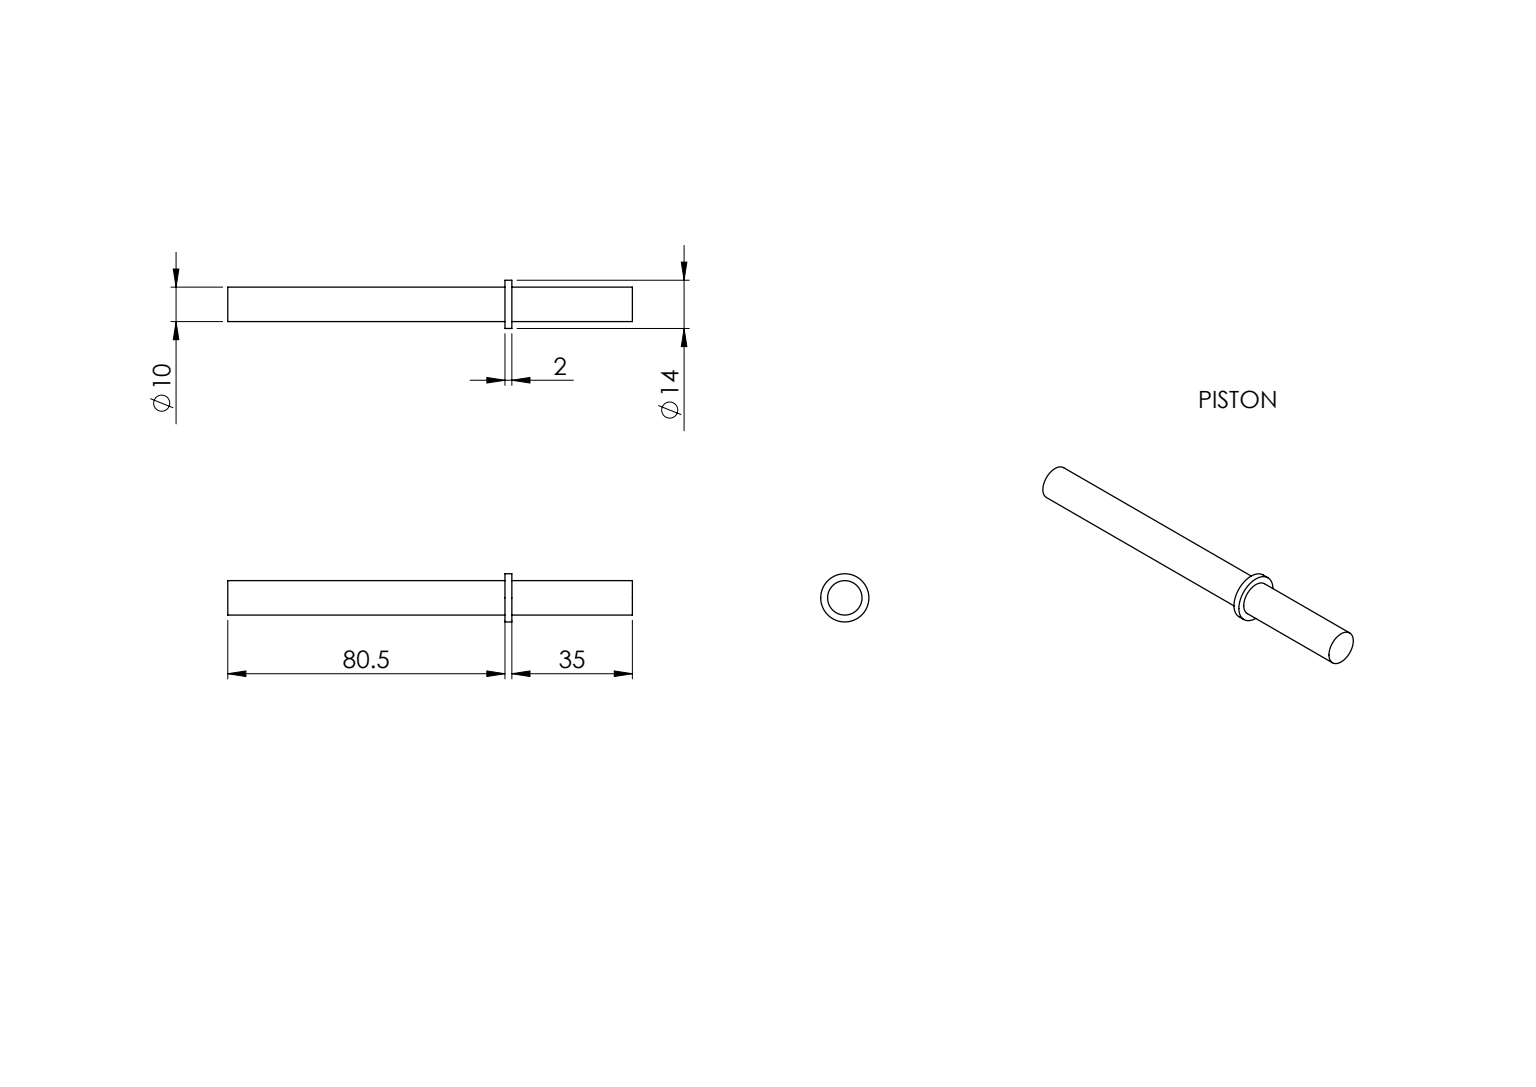
ISO-10303-21;
HEADER;
FILE_DESCRIPTION (('STEP AP214'),
    '1' );
FILE_NAME ('piston.step',
    '2026-10-27T14:18:53',
    ( '' ),
    ( '' ),
    'SwSTEP 2.0',
    'SolidWorks 2026',
    '' );
FILE_SCHEMA (( 'AUTOMOTIVE_DESIGN' ));
ENDSEC;

DATA;
#2=PLANE ( 'NONE',  #2825 ) ;
#50=DIRECTION ( 'NONE',  ( -1.000000000000000000, -0.000000000000000000, -0.000000000000000000 ) ) ;
#53=( NAMED_UNIT ( * ) PLANE_ANGLE_UNIT ( ) SI_UNIT ( $, .RADIAN. ) );
#122=CARTESIAN_POINT ( 'NONE',  ( 135.4999999999999716, 0.000000000000000000, 0.000000000000000000 ) ) ;
#126=MANIFOLD_SOLID_BREP ( 'Boss-Extrude2', #2558 ) ;
#155=ORIENTED_EDGE ( 'NONE', *, *, #5293, .T. ) ;
#159=EDGE_CURVE ( 'NONE', #4312, #626, #169, .T. ) ;
#169=LINE ( 'NONE', #5681, #675 ) ;
#172=DIRECTION ( 'NONE',  ( 0.000000000000000000, 0.000000000000000000, -1.000000000000000000 ) ) ;
#214=CARTESIAN_POINT ( 'NONE',  ( 137.4999999999999716, 0.000000000000000000, 5.000000000000000000 ) ) ;
#218=AXIS2_PLACEMENT_3D ( 'NONE', #3417, #2963, #2469 ) ;
#223=AXIS2_PLACEMENT_3D ( 'NONE', #4631, #50, #5962 ) ;
#241=SHAPE_DEFINITION_REPRESENTATION ( #544, #4225 ) ;
#261=ORIENTED_EDGE ( 'NONE', *, *, #932, .T. ) ;
#264=DIRECTION ( 'NONE',  ( -1.000000000000000000, -0.000000000000000000, -0.000000000000000000 ) ) ;
#265=ORIENTED_EDGE ( 'NONE', *, *, #3879, .F. ) ;
#267=CARTESIAN_POINT ( 'NONE',  ( 196.6421356237309510, 0.000000000000000000, 5.000000000000000000 ) ) ;
#289=DIRECTION ( 'NONE',  ( 0.000000000000000000, 0.000000000000000000, 1.000000000000000000 ) ) ;
#334=ADVANCED_FACE ( 'NONE', ( #4537 ), #4626, .F. ) ;
#384=ORIENTED_EDGE ( 'NONE', *, *, #5078, .T. ) ;
#395=EDGE_LOOP ( 'NONE', ( #4054, #2100 ) ) ;
#411=VECTOR ( 'NONE', #264, 1000.000000000000000 ) ;
#430=( LENGTH_UNIT ( ) NAMED_UNIT ( * ) SI_UNIT ( .MILLI., .METRE. ) );
#451=PLANE ( 'NONE',  #1857 ) ;
#456=VECTOR ( 'NONE', #5335, 1000.000000000000000 ) ;
#462=CARTESIAN_POINT ( 'NONE',  ( 172.5000000000000284, 15.00000000000000000, 75.00000000000001421 ) ) ;
#466=DIRECTION ( 'NONE',  ( -1.000000000000000000, 0.000000000000000000, 0.000000000000000000 ) ) ;
#478=CARTESIAN_POINT ( 'NONE',  ( 55.00000000000000711, 0.000000000000000000, 5.000000000000000000 ) ) ;
#544=PRODUCT_DEFINITION_SHAPE ( 'NONE', 'NONE',  #3311 ) ;
#575=AXIS2_PLACEMENT_3D ( 'NONE', #1998, #3850, #3404 ) ;
#590=AXIS2_PLACEMENT_3D ( 'NONE', #4311, #4369, #5694 ) ;
#626=VERTEX_POINT ( 'NONE', #3463 ) ;
#647=ORIENTED_EDGE ( 'NONE', *, *, #1643, .T. ) ;
#663=AXIS2_PLACEMENT_3D ( 'NONE', #4941, #4491, #775 ) ;
#667=DIRECTION ( 'NONE',  ( 1.000000000000000000, 0.000000000000000000, 0.000000000000000000 ) ) ;
#675=VECTOR ( 'NONE', #3854, 1000.000000000000000 ) ;
#676=AXIS2_PLACEMENT_3D ( 'NONE', #3452, #3515, #5369 ) ;
#749=CARTESIAN_POINT ( 'NONE',  ( 137.4999999999999716, 8.572527594031473190E-16, 7.000000000000000000 ) ) ;
#775=DIRECTION ( 'NONE',  ( 0.000000000000000000, 0.000000000000000000, -1.000000000000000000 ) ) ;
#780=DIRECTION ( 'NONE',  ( 1.000000000000000000, -0.000000000000000000, -0.000000000000000000 ) ) ;
#795=VECTOR ( 'NONE', #780, 1000.000000000000000 ) ;
#810=ADVANCED_FACE ( 'NONE', ( #4064 ), #3617, .T. ) ;
#817=( NAMED_UNIT ( * ) PLANE_ANGLE_UNIT ( ) SI_UNIT ( $, .RADIAN. ) );
#852=ORIENTED_EDGE ( 'NONE', *, *, #5084, .T. ) ;
#873=CYLINDRICAL_SURFACE ( 'NONE', #5492, 7.000000000000000000 ) ;
#920=FACE_OUTER_BOUND ( 'NONE', #5008, .T. ) ;
#926=AXIS2_PLACEMENT_3D ( 'NONE', #3342, #2851, #4711 ) ;
#927=FACE_OUTER_BOUND ( 'NONE', #3682, .T. ) ;
#932=EDGE_CURVE ( 'NONE', #3440, #5157, #3043, .T. ) ;
#936=EDGE_LOOP ( 'NONE', ( #4735, #3724 ) ) ;
#953=CARTESIAN_POINT ( 'NONE',  ( 55.00000000000000711, 0.000000000000000000, 0.000000000000000000 ) ) ;
#961=( GEOMETRIC_REPRESENTATION_CONTEXT ( 3 ) GLOBAL_UNCERTAINTY_ASSIGNED_CONTEXT ( ( #1965 ) ) GLOBAL_UNIT_ASSIGNED_CONTEXT ( ( #2755, #53, #2314 ) ) REPRESENTATION_CONTEXT ( 'NONE', 'WORKASPACE' ) );
#976=EDGE_CURVE ( 'NONE', #626, #5459, #5968, .T. ) ;
#983=AXIS2_PLACEMENT_3D ( 'NONE', #5013, #5074, #3743 ) ;
#1135=CARTESIAN_POINT ( 'NONE',  ( 135.4999999999999716, 0.000000000000000000, 5.000000000000000000 ) ) ;
#1138=ORIENTED_EDGE ( 'NONE', *, *, #976, .T. ) ;
#1149=EDGE_LOOP ( 'NONE', ( #265, #5106 ) ) ;
#1172=CIRCLE ( 'NONE', #218, 5.000000000000000000 ) ;
#1176=( LENGTH_UNIT ( ) NAMED_UNIT ( * ) SI_UNIT ( .MILLI., .METRE. ) );
#1185=STYLED_ITEM ( 'NONE', ( #4986 ), #3198 ) ;
#1251=EDGE_LOOP ( 'NONE', ( #5497, #155, #2860, #3324 ) ) ;
#1262=UNCERTAINTY_MEASURE_WITH_UNIT (LENGTH_MEASURE( 1.000000000000000082E-05 ), #1176, 'distance_accuracy_value', 'NONE');
#1265=ORIENTED_EDGE ( 'NONE', *, *, #5682, .T. ) ;
#1285=ORIENTED_EDGE ( 'NONE', *, *, #1568, .F. ) ;
#1305=CARTESIAN_POINT ( 'NONE',  ( 135.4999999999999716, 0.000000000000000000, 0.000000000000000000 ) ) ;
#1310=ORIENTED_EDGE ( 'NONE', *, *, #5372, .T. ) ;
#1320=ADVANCED_FACE ( 'NONE', ( #5046 ), #873, .T. ) ;
#1327=VERTEX_POINT ( 'NONE', #478 ) ;
#1332=CARTESIAN_POINT ( 'NONE',  ( 172.5000000000000284, 0.000000000000000000, 5.000000000000000000 ) ) ;
#1402=CYLINDRICAL_SURFACE ( 'NONE', #4867, 5.000000000000000000 ) ;
#1446=AXIS2_PLACEMENT_3D ( 'NONE', #3748, #3337, #5692 ) ;
#1460=VECTOR ( 'NONE', #4573, 1000.000000000000000 ) ;
#1469=CARTESIAN_POINT ( 'NONE',  ( 135.4999999999999716, 0.000000000000000000, 0.000000000000000000 ) ) ;
#1525=DIRECTION ( 'NONE',  ( 1.000000000000000000, 0.000000000000000000, 0.000000000000000000 ) ) ;
#1568=EDGE_CURVE ( 'NONE', #2772, #5459, #5846, .T. ) ;
#1593=CARTESIAN_POINT ( 'NONE',  ( 137.4999999999999716, 0.000000000000000000, -7.000000000000000000 ) ) ;
#1639=ORIENTED_EDGE ( 'NONE', *, *, #2435, .T. ) ;
#1643=EDGE_CURVE ( 'NONE', #1327, #4518, #3174, .T. ) ;
#1728=DIRECTION ( 'NONE',  ( 0.000000000000000000, 0.000000000000000000, -1.000000000000000000 ) ) ;
#1800=DIRECTION ( 'NONE',  ( 0.000000000000000000, 0.000000000000000000, 1.000000000000000000 ) ) ;
#1809=FACE_OUTER_BOUND ( 'NONE', #395, .T. ) ;
#1857=AXIS2_PLACEMENT_3D ( 'NONE', #953, #2320, #2380 ) ;
#1867=DIRECTION ( 'NONE',  ( 0.000000000000000000, 0.000000000000000000, 1.000000000000000000 ) ) ;
#1885=CARTESIAN_POINT ( 'NONE',  ( 172.5000000000000284, 0.000000000000000000, 0.000000000000000000 ) ) ;
#1956=MECHANICAL_DESIGN_GEOMETRIC_PRESENTATION_REPRESENTATION('',(#1185),#4684);
#1965=UNCERTAINTY_MEASURE_WITH_UNIT (LENGTH_MEASURE( 1.000000000000000082E-05 ), #2755, 'distance_accuracy_value', 'NONE');
#1998=CARTESIAN_POINT ( 'NONE',  ( 137.4999999999999716, 0.000000000000000000, 0.000000000000000000 ) ) ;
#2001=ORIENTED_EDGE ( 'NONE', *, *, #5660, .F. ) ;
#2015=PLANE ( 'NONE',  #676 ) ;
#2023=( NAMED_UNIT ( * ) SI_UNIT ( $, .STERADIAN. ) SOLID_ANGLE_UNIT ( ) );
#2100=ORIENTED_EDGE ( 'NONE', *, *, #3397, .F. ) ;
#2142=FACE_OUTER_BOUND ( 'NONE', #1251, .T. ) ;
#2147=( NAMED_UNIT ( * ) SI_UNIT ( $, .STERADIAN. ) SOLID_ANGLE_UNIT ( ) );
#2149=AXIS2_PLACEMENT_3D ( 'NONE', #4002, #5456, #3158 ) ;
#2171=LINE ( 'NONE', #4021, #1460 ) ;
#2198=DIRECTION ( 'NONE',  ( -1.000000000000000000, 0.000000000000000000, 0.000000000000000000 ) ) ;
#2217=DIRECTION ( 'NONE',  ( 0.000000000000000000, 0.000000000000000000, 1.000000000000000000 ) ) ;
#2226=EDGE_LOOP ( 'NONE', ( #852, #1310, #3329, #3767 ) ) ;
#2242=AXIS2_PLACEMENT_3D ( 'NONE', #122, #2540, #4341 ) ;
#2290=DIRECTION ( 'NONE',  ( 0.000000000000000000, 0.000000000000000000, 1.000000000000000000 ) ) ;
#2311=FACE_OUTER_BOUND ( 'NONE', #5227, .T. ) ;
#2312=VERTEX_POINT ( 'NONE', #4606 ) ;
#2314=( NAMED_UNIT ( * ) SI_UNIT ( $, .STERADIAN. ) SOLID_ANGLE_UNIT ( ) );
#2320=DIRECTION ( 'NONE',  ( 1.000000000000000000, 0.000000000000000000, 0.000000000000000000 ) ) ;
#2380=DIRECTION ( 'NONE',  ( 0.000000000000000000, 0.000000000000000000, -1.000000000000000000 ) ) ;
#2383=ORIENTED_EDGE ( 'NONE', *, *, #5393, .F. ) ;
#2435=EDGE_CURVE ( 'NONE', #5618, #3394, #3004, .T. ) ;
#2454=DIRECTION ( 'NONE',  ( -1.000000000000000000, 0.000000000000000000, 0.000000000000000000 ) ) ;
#2457=ORIENTED_EDGE ( 'NONE', *, *, #4055, .T. ) ;
#2469=DIRECTION ( 'NONE',  ( 0.000000000000000000, 0.000000000000000000, 1.000000000000000000 ) ) ;
#2503=ORIENTED_EDGE ( 'NONE', *, *, #932, .F. ) ;
#2526=CARTESIAN_POINT ( 'NONE',  ( 55.00000000000000711, 0.000000000000000000, 0.000000000000000000 ) ) ;
#2531=CARTESIAN_POINT ( 'NONE',  ( 135.4999999999999716, 0.000000000000000000, -7.000000000000000000 ) ) ;
#2534=PRODUCT_CONTEXT ( 'NONE', #2846, 'mechanical' ) ;
#2540=DIRECTION ( 'NONE',  ( -1.000000000000000000, 0.000000000000000000, 0.000000000000000000 ) ) ;
#2558=CLOSED_SHELL ( 'NONE', ( #4050, #810, #2681, #5719, #4047, #1320, #5759, #2881, #334, #5678 ) ) ;
#2599=SURFACE_STYLE_FILL_AREA ( #4527 ) ;
#2617=CARTESIAN_POINT ( 'NONE',  ( 135.4999999999999716, 8.572527594031473190E-16, 7.000000000000000000 ) ) ;
#2637=DIRECTION ( 'NONE',  ( 1.000000000000000000, -0.000000000000000000, -0.000000000000000000 ) ) ;
#2681=ADVANCED_FACE ( 'NONE', ( #5662 ), #5954, .T. ) ;
#2743=AXIS2_PLACEMENT_3D ( 'NONE', #1305, #3165, #1728 ) ;
#2755=( LENGTH_UNIT ( ) NAMED_UNIT ( * ) SI_UNIT ( .MILLI., .METRE. ) );
#2772=VERTEX_POINT ( 'NONE', #1332 ) ;
#2802=EDGE_LOOP ( 'NONE', ( #3718, #1138 ) ) ;
#2809=FACE_BOUND ( 'NONE', #3116, .T. ) ;
#2825=AXIS2_PLACEMENT_3D ( 'NONE', #1469, #4151, #1867 ) ;
#2827=AXIS2_PLACEMENT_3D ( 'NONE', #4019, #4422, #289 ) ;
#2846=APPLICATION_CONTEXT ( 'automotive_design' ) ;
#2851=DIRECTION ( 'NONE',  ( -1.000000000000000000, 0.000000000000000000, 0.000000000000000000 ) ) ;
#2860=ORIENTED_EDGE ( 'NONE', *, *, #1568, .T. ) ;
#2881=ADVANCED_FACE ( 'NONE', ( #5338, #2968 ), #2015, .F. ) ;
#2949=VERTEX_POINT ( 'NONE', #1135 ) ;
#2963=DIRECTION ( 'NONE',  ( -1.000000000000000000, 0.000000000000000000, 0.000000000000000000 ) ) ;
#2968=FACE_OUTER_BOUND ( 'NONE', #1149, .T. ) ;
#3004=CIRCLE ( 'NONE', #575, 7.000000000000000000 ) ;
#3039=( GEOMETRIC_REPRESENTATION_CONTEXT ( 3 ) GLOBAL_UNCERTAINTY_ASSIGNED_CONTEXT ( ( #1262 ) ) GLOBAL_UNIT_ASSIGNED_CONTEXT ( ( #1176, #3521, #2023 ) ) REPRESENTATION_CONTEXT ( 'NONE', 'WORKASPACE' ) );
#3040=ORIENTED_EDGE ( 'NONE', *, *, #5426, .T. ) ;
#3043=CIRCLE ( 'NONE', #5277, 7.000000000000000000 ) ;
#3087=UNCERTAINTY_MEASURE_WITH_UNIT (LENGTH_MEASURE( 1.000000000000000082E-05 ), #430, 'distance_accuracy_value', 'NONE');
#3093=SURFACE_SIDE_STYLE ('',( #2599 ) ) ;
#3116=EDGE_LOOP ( 'NONE', ( #3340, #4294 ) ) ;
#3118=VECTOR ( 'NONE', #5066, 1000.000000000000000 ) ;
#3158=DIRECTION ( 'NONE',  ( 0.000000000000000000, 0.000000000000000000, 1.000000000000000000 ) ) ;
#3165=DIRECTION ( 'NONE',  ( 1.000000000000000000, -0.000000000000000000, -0.000000000000000000 ) ) ;
#3174=CIRCLE ( 'NONE', #663, 5.000000000000000000 ) ;
#3187=CARTESIAN_POINT ( 'NONE',  ( 135.4999999999999716, 0.000000000000000000, -7.000000000000000000 ) ) ;
#3191=SHAPE_REPRESENTATION_RELATIONSHIP ( 'NONE' , 'NONE' ,  #4225, #3198 ) ;
#3198=ADVANCED_BREP_SHAPE_REPRESENTATION ( '', ( #126, #5080 ), #3039 ) ;
#3207=CYLINDRICAL_SURFACE ( 'NONE', #223, 5.000000000000000000 ) ;
#3210=CARTESIAN_POINT ( 'NONE',  ( 135.4999999999999716, 8.572527594031473190E-16, 7.000000000000000000 ) ) ;
#3222=FILL_AREA_STYLE_COLOUR ( '', #4202 ) ;
#3264=ORIENTED_EDGE ( 'NONE', *, *, #5393, .T. ) ;
#3311=PRODUCT_DEFINITION ( 'UNKNOWN', '', #4599, #5937 ) ;
#3324=ORIENTED_EDGE ( 'NONE', *, *, #976, .F. ) ;
#3329=ORIENTED_EDGE ( 'NONE', *, *, #3397, .T. ) ;
#3337=DIRECTION ( 'NONE',  ( -1.000000000000000000, -0.000000000000000000, -0.000000000000000000 ) ) ;
#3340=ORIENTED_EDGE ( 'NONE', *, *, #5084, .F. ) ;
#3342=CARTESIAN_POINT ( 'NONE',  ( 137.4999999999999716, 0.000000000000000000, 0.000000000000000000 ) ) ;
#3352=ORIENTED_EDGE ( 'NONE', *, *, #3879, .T. ) ;
#3394=VERTEX_POINT ( 'NONE', #1593 ) ;
#3397=EDGE_CURVE ( 'NONE', #4518, #1327, #5153, .T. ) ;
#3404=DIRECTION ( 'NONE',  ( 0.000000000000000000, 0.000000000000000000, 1.000000000000000000 ) ) ;
#3414=EDGE_LOOP ( 'NONE', ( #2503, #3264, #1639, #2001 ) ) ;
#3417=CARTESIAN_POINT ( 'NONE',  ( 135.4999999999999716, 0.000000000000000000, 0.000000000000000000 ) ) ;
#3440=VERTEX_POINT ( 'NONE', #2617 ) ;
#3452=CARTESIAN_POINT ( 'NONE',  ( 137.4999999999999716, 0.000000000000000000, 0.000000000000000000 ) ) ;
#3463=CARTESIAN_POINT ( 'NONE',  ( 137.4999999999999716, 6.123233995736766282E-16, -5.000000000000000000 ) ) ;
#3515=DIRECTION ( 'NONE',  ( -1.000000000000000000, 0.000000000000000000, 0.000000000000000000 ) ) ;
#3521=( NAMED_UNIT ( * ) PLANE_ANGLE_UNIT ( ) SI_UNIT ( $, .RADIAN. ) );
#3527=CARTESIAN_POINT ( 'NONE',  ( 0.000000000000000000, 0.000000000000000000, 0.000000000000000000 ) ) ;
#3617=CYLINDRICAL_SURFACE ( 'NONE', #2743, 7.000000000000000000 ) ;
#3631=CARTESIAN_POINT ( 'NONE',  ( 172.5000000000000284, 0.000000000000000000, 0.000000000000000000 ) ) ;
#3657=LINE ( 'NONE', #3210, #3118 ) ;
#3682=EDGE_LOOP ( 'NONE', ( #1265, #261 ) ) ;
#3699=AXIS2_PLACEMENT_3D ( 'NONE', #3631, #2198, #4543 ) ;
#3718=ORIENTED_EDGE ( 'NONE', *, *, #4697, .T. ) ;
#3724=ORIENTED_EDGE ( 'NONE', *, *, #5293, .F. ) ;
#3743=DIRECTION ( 'NONE',  ( 0.000000000000000000, 0.000000000000000000, 1.000000000000000000 ) ) ;
#3748=CARTESIAN_POINT ( 'NONE',  ( 196.6421356237309510, 0.000000000000000000, 0.000000000000000000 ) ) ;
#3749=CARTESIAN_POINT ( 'NONE',  ( 55.00000000000000711, 6.123233995736766282E-16, -5.000000000000000000 ) ) ;
#3767=ORIENTED_EDGE ( 'NONE', *, *, #5078, .F. ) ;
#3787=CIRCLE ( 'NONE', #4771, 5.000000000000000000 ) ;
#3799=ORIENTED_EDGE ( 'NONE', *, *, #4697, .F. ) ;
#3850=DIRECTION ( 'NONE',  ( -1.000000000000000000, 0.000000000000000000, 0.000000000000000000 ) ) ;
#3854=DIRECTION ( 'NONE',  ( -1.000000000000000000, -0.000000000000000000, -0.000000000000000000 ) ) ;
#3879=EDGE_CURVE ( 'NONE', #3394, #5618, #4192, .T. ) ;
#3986=ORIENTED_EDGE ( 'NONE', *, *, #5682, .F. ) ;
#4002=CARTESIAN_POINT ( 'NONE',  ( 196.6421356237309510, 0.000000000000000000, 0.000000000000000000 ) ) ;
#4019=CARTESIAN_POINT ( 'NONE',  ( 137.4999999999999716, 0.000000000000000000, 0.000000000000000000 ) ) ;
#4021=CARTESIAN_POINT ( 'NONE',  ( 196.6421356237309510, 6.123233995736766282E-16, -5.000000000000000000 ) ) ;
#4047=ADVANCED_FACE ( 'NONE', ( #2311 ), #3207, .T. ) ;
#4050=ADVANCED_FACE ( 'NONE', ( #920 ), #1402, .T. ) ;
#4054=ORIENTED_EDGE ( 'NONE', *, *, #1643, .F. ) ;
#4055=EDGE_CURVE ( 'NONE', #2772, #4312, #3787, .T. ) ;
#4064=FACE_OUTER_BOUND ( 'NONE', #3414, .T. ) ;
#4078=CIRCLE ( 'NONE', #590, 5.000000000000000000 ) ;
#4099=EDGE_LOOP ( 'NONE', ( #2383, #3986, #5294, #3352 ) ) ;
#4151=DIRECTION ( 'NONE',  ( -1.000000000000000000, 0.000000000000000000, 0.000000000000000000 ) ) ;
#4192=CIRCLE ( 'NONE', #2827, 7.000000000000000000 ) ;
#4202=COLOUR_RGB ( '',0.8941176470588234615, 0.8941176470588234615, 0.8941176470588234615 ) ;
#4208=AXIS2_PLACEMENT_3D ( 'NONE', #462, #5557, #2217 ) ;
#4225=SHAPE_REPRESENTATION ( 'piston', ( #5080 ), #3039 ) ;
#4294=ORIENTED_EDGE ( 'NONE', *, *, #5426, .F. ) ;
#4311=CARTESIAN_POINT ( 'NONE',  ( 137.4999999999999716, 0.000000000000000000, 0.000000000000000000 ) ) ;
#4312=VERTEX_POINT ( 'NONE', #5909 ) ;
#4341=DIRECTION ( 'NONE',  ( 0.000000000000000000, 0.000000000000000000, 1.000000000000000000 ) ) ;
#4369=DIRECTION ( 'NONE',  ( -1.000000000000000000, 0.000000000000000000, 0.000000000000000000 ) ) ;
#4422=DIRECTION ( 'NONE',  ( -1.000000000000000000, 0.000000000000000000, 0.000000000000000000 ) ) ;
#4467=MECHANICAL_DESIGN_GEOMETRIC_PRESENTATION_REPRESENTATION('',(#4950),#961);
#4491=DIRECTION ( 'NONE',  ( 1.000000000000000000, 0.000000000000000000, 0.000000000000000000 ) ) ;
#4495=LINE ( 'NONE', #3187, #795 ) ;
#4499=DIRECTION ( 'NONE',  ( 0.000000000000000000, 0.000000000000000000, -1.000000000000000000 ) ) ;
#4518=VERTEX_POINT ( 'NONE', #3749 ) ;
#4527=FILL_AREA_STYLE ('',( #3222 ) ) ;
#4537=FACE_OUTER_BOUND ( 'NONE', #936, .T. ) ;
#4543=DIRECTION ( 'NONE',  ( 0.000000000000000000, 0.000000000000000000, 1.000000000000000000 ) ) ;
#4573=DIRECTION ( 'NONE',  ( -1.000000000000000000, -0.000000000000000000, -0.000000000000000000 ) ) ;
#4599=PRODUCT_DEFINITION_FORMATION_WITH_SPECIFIED_SOURCE ( 'ANY', '', #4847, .NOT_KNOWN. ) ;
#4606=CARTESIAN_POINT ( 'NONE',  ( 135.4999999999999716, 6.123233995736766282E-16, -5.000000000000000000 ) ) ;
#4626=PLANE ( 'NONE',  #4208 ) ;
#4631=CARTESIAN_POINT ( 'NONE',  ( 196.6421356237309510, 0.000000000000000000, 0.000000000000000000 ) ) ;
#4672=CIRCLE ( 'NONE', #2242, 5.000000000000000000 ) ;
#4681=CARTESIAN_POINT ( 'NONE',  ( 135.4999999999999716, 0.000000000000000000, 0.000000000000000000 ) ) ;
#4684=( GEOMETRIC_REPRESENTATION_CONTEXT ( 3 ) GLOBAL_UNCERTAINTY_ASSIGNED_CONTEXT ( ( #3087 ) ) GLOBAL_UNIT_ASSIGNED_CONTEXT ( ( #430, #817, #2147 ) ) REPRESENTATION_CONTEXT ( 'NONE', 'WORKASPACE' ) );
#4697=EDGE_CURVE ( 'NONE', #5459, #626, #4078, .T. ) ;
#4711=DIRECTION ( 'NONE',  ( 0.000000000000000000, 0.000000000000000000, 1.000000000000000000 ) ) ;
#4735=ORIENTED_EDGE ( 'NONE', *, *, #4055, .F. ) ;
#4753=LINE ( 'NONE', #4883, #411 ) ;
#4769=CIRCLE ( 'NONE', #3699, 5.000000000000000000 ) ;
#4771=AXIS2_PLACEMENT_3D ( 'NONE', #1885, #466, #1800 ) ;
#4831=DIRECTION ( 'NONE',  ( 0.000000000000000000, 0.000000000000000000, 1.000000000000000000 ) ) ;
#4847=PRODUCT ( 'piston', 'piston', '', ( #2534 ) ) ;
#4867=AXIS2_PLACEMENT_3D ( 'NONE', #5093, #5145, #2290 ) ;
#4883=CARTESIAN_POINT ( 'NONE',  ( 196.6421356237309510, 0.000000000000000000, 5.000000000000000000 ) ) ;
#4935=ORIENTED_EDGE ( 'NONE', *, *, #5372, .F. ) ;
#4941=CARTESIAN_POINT ( 'NONE',  ( 55.00000000000000711, 0.000000000000000000, 0.000000000000000000 ) ) ;
#4943=APPLICATION_CONTEXT ( 'automotive_design' ) ;
#4950=STYLED_ITEM('',(#6013),#126);
#4986=PRESENTATION_STYLE_ASSIGNMENT (( #5045 ) ) ;
#5008=EDGE_LOOP ( 'NONE', ( #2457, #5580, #3799, #1285 ) ) ;
#5013=CARTESIAN_POINT ( 'NONE',  ( 135.4999999999999716, 0.000000000000000000, 0.000000000000000000 ) ) ;
#5045=SURFACE_STYLE_USAGE ( .BOTH. , #3093 ) ;
#5046=FACE_OUTER_BOUND ( 'NONE', #4099, .T. ) ;
#5066=DIRECTION ( 'NONE',  ( 1.000000000000000000, -0.000000000000000000, -0.000000000000000000 ) ) ;
#5074=DIRECTION ( 'NONE',  ( -1.000000000000000000, 0.000000000000000000, 0.000000000000000000 ) ) ;
#5078=EDGE_CURVE ( 'NONE', #2949, #1327, #4753, .T. ) ;
#5080=AXIS2_PLACEMENT_3D ( 'NONE', #3527, #4831, #667 ) ;
#5084=EDGE_CURVE ( 'NONE', #2949, #2312, #1172, .T. ) ;
#5093=CARTESIAN_POINT ( 'NONE',  ( 196.6421356237309510, 0.000000000000000000, 0.000000000000000000 ) ) ;
#5106=ORIENTED_EDGE ( 'NONE', *, *, #2435, .F. ) ;
#5145=DIRECTION ( 'NONE',  ( -1.000000000000000000, -0.000000000000000000, -0.000000000000000000 ) ) ;
#5153=CIRCLE ( 'NONE', #5246, 5.000000000000000000 ) ;
#5157=VERTEX_POINT ( 'NONE', #2531 ) ;
#5215=DIRECTION ( 'NONE',  ( 0.000000000000000000, 0.000000000000000000, 1.000000000000000000 ) ) ;
#5227=EDGE_LOOP ( 'NONE', ( #4935, #3040, #384, #647 ) ) ;
#5246=AXIS2_PLACEMENT_3D ( 'NONE', #2526, #1525, #172 ) ;
#5277=AXIS2_PLACEMENT_3D ( 'NONE', #4681, #2454, #5215 ) ;
#5293=EDGE_CURVE ( 'NONE', #4312, #2772, #4769, .T. ) ;
#5294=ORIENTED_EDGE ( 'NONE', *, *, #5660, .T. ) ;
#5335=DIRECTION ( 'NONE',  ( -1.000000000000000000, -0.000000000000000000, -0.000000000000000000 ) ) ;
#5338=FACE_BOUND ( 'NONE', #2802, .T. ) ;
#5369=DIRECTION ( 'NONE',  ( 0.000000000000000000, 0.000000000000000000, 1.000000000000000000 ) ) ;
#5372=EDGE_CURVE ( 'NONE', #2312, #4518, #2171, .T. ) ;
#5393=EDGE_CURVE ( 'NONE', #3440, #5618, #3657, .T. ) ;
#5426=EDGE_CURVE ( 'NONE', #2312, #2949, #4672, .T. ) ;
#5456=DIRECTION ( 'NONE',  ( -1.000000000000000000, -0.000000000000000000, -0.000000000000000000 ) ) ;
#5459=VERTEX_POINT ( 'NONE', #214 ) ;
#5492=AXIS2_PLACEMENT_3D ( 'NONE', #5549, #2637, #4499 ) ;
#5497=ORIENTED_EDGE ( 'NONE', *, *, #159, .F. ) ;
#5549=CARTESIAN_POINT ( 'NONE',  ( 135.4999999999999716, 0.000000000000000000, 0.000000000000000000 ) ) ;
#5557=DIRECTION ( 'NONE',  ( -1.000000000000000000, 0.000000000000000000, 0.000000000000000000 ) ) ;
#5580=ORIENTED_EDGE ( 'NONE', *, *, #159, .T. ) ;
#5618=VERTEX_POINT ( 'NONE', #749 ) ;
#5631=CIRCLE ( 'NONE', #983, 7.000000000000000000 ) ;
#5660=EDGE_CURVE ( 'NONE', #5157, #3394, #4495, .T. ) ;
#5662=FACE_OUTER_BOUND ( 'NONE', #2226, .T. ) ;
#5678=ADVANCED_FACE ( 'NONE', ( #2142 ), #5899, .T. ) ;
#5681=CARTESIAN_POINT ( 'NONE',  ( 196.6421356237309510, 6.123233995736766282E-16, -5.000000000000000000 ) ) ;
#5682=EDGE_CURVE ( 'NONE', #5157, #3440, #5631, .T. ) ;
#5692=DIRECTION ( 'NONE',  ( 0.000000000000000000, 0.000000000000000000, 1.000000000000000000 ) ) ;
#5694=DIRECTION ( 'NONE',  ( 0.000000000000000000, 0.000000000000000000, 1.000000000000000000 ) ) ;
#5719=ADVANCED_FACE ( 'NONE', ( #1809 ), #451, .F. ) ;
#5759=ADVANCED_FACE ( 'NONE', ( #2809, #927 ), #2, .T. ) ;
#5846=LINE ( 'NONE', #267, #456 ) ;
#5899=CYLINDRICAL_SURFACE ( 'NONE', #2149, 5.000000000000000000 ) ;
#5909=CARTESIAN_POINT ( 'NONE',  ( 172.5000000000000284, 6.123233995736766282E-16, -5.000000000000000000 ) ) ;
#5937=PRODUCT_DEFINITION_CONTEXT ( 'detailed design', #4943, 'design' ) ;
#5954=CYLINDRICAL_SURFACE ( 'NONE', #1446, 5.000000000000000000 ) ;
#5962=DIRECTION ( 'NONE',  ( 0.000000000000000000, 0.000000000000000000, 1.000000000000000000 ) ) ;
#5968=CIRCLE ( 'NONE', #926, 5.000000000000000000 ) ;
#6007=COLOUR_RGB('Sky Blue',0.24,0.69,0.87);
#6008=FILL_AREA_STYLE_COLOUR('',#6007);
#6009=FILL_AREA_STYLE('',(#6008));
#6010=SURFACE_STYLE_FILL_AREA(#6009);
#6011=SURFACE_SIDE_STYLE('',(#6010));
#6012=SURFACE_STYLE_USAGE(.BOTH.,#6011);
#6013=PRESENTATION_STYLE_ASSIGNMENT((#6012));
ENDSEC;
END-ISO-10303-21;
